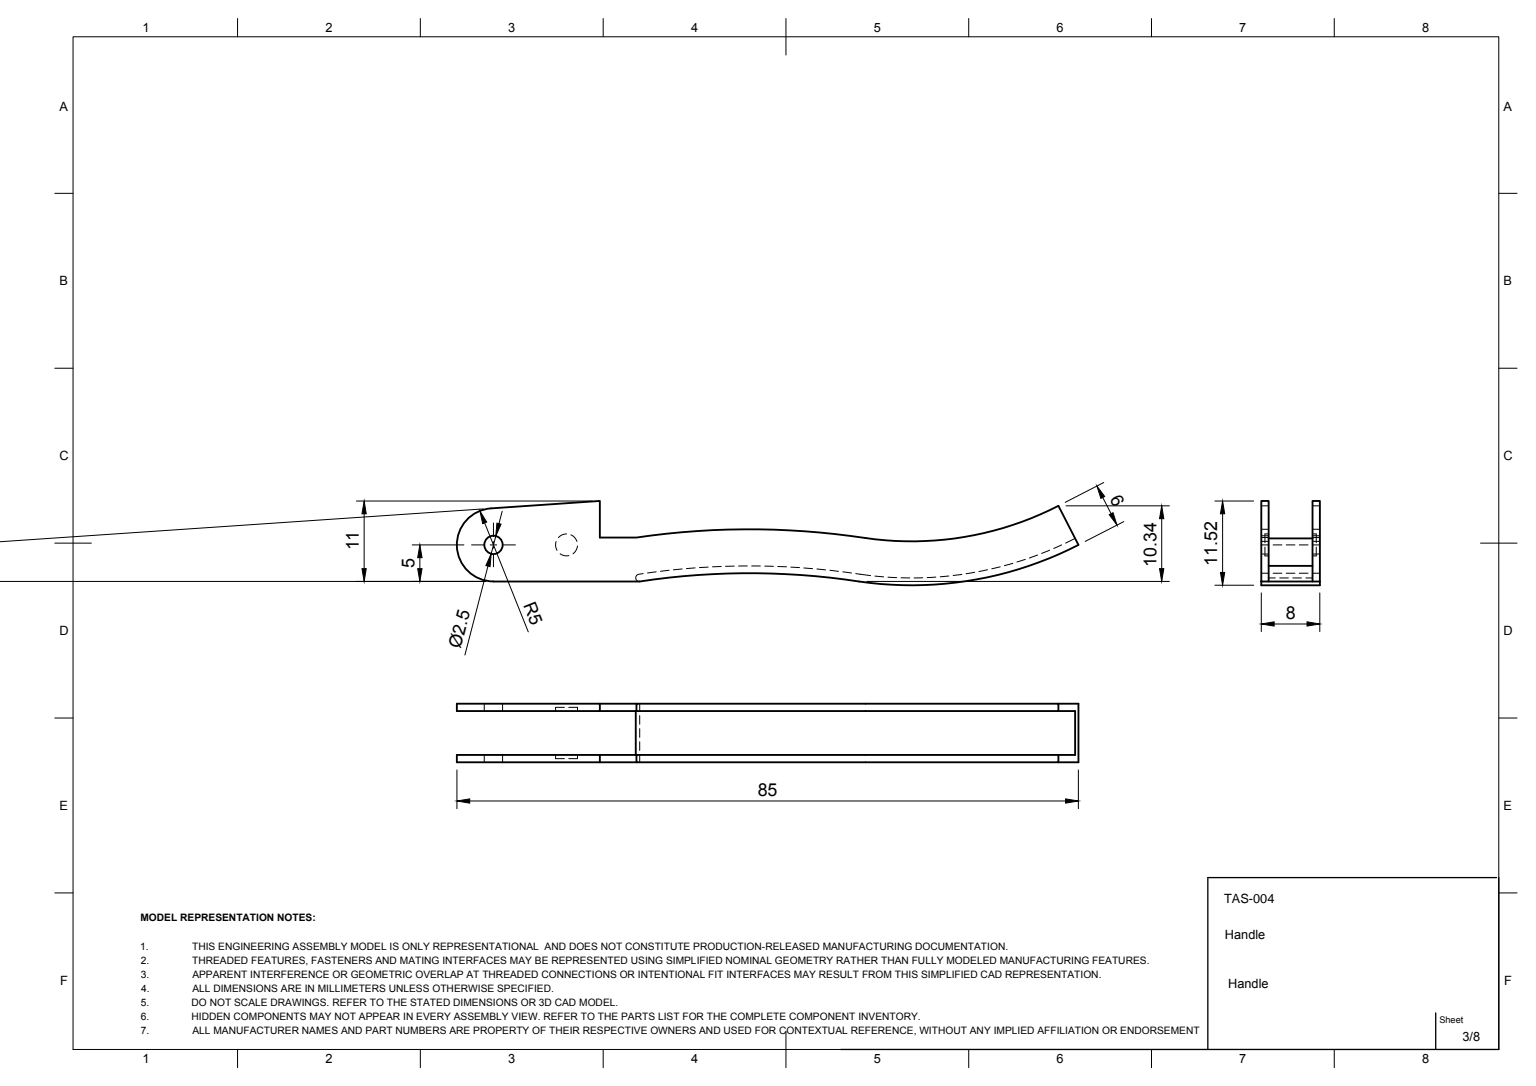
ISO-10303-21;
HEADER;
/* Generated by software containing ST-Developer
 * from STEP Tools, Inc. (www.steptools.com) 
 */

FILE_DESCRIPTION(
/* description */ ('STEP AP214'),
/* implementation_level */ '2;1');

FILE_NAME(
/* name */ 'Handle.step',
/* time_stamp */ '2026-11-04T19:48:07-08:00',
/* author */ (''),
/* organization */ (''),
/* preprocessor_version */ 'ST-DEVELOPER v20.2',
/* originating_system */ 'Autodesk Translation Framework v15.17.0.0',
/* authorisation */ '');

FILE_SCHEMA (('AUTOMOTIVE_DESIGN { 1 0 10303 214 3 1 1 }'));
ENDSEC;

DATA;
#10=MECHANICAL_DESIGN_GEOMETRIC_PRESENTATION_REPRESENTATION('',(#59),#9561);
#47=SHAPE_REPRESENTATION_RELATIONSHIP('SRR','None',#9587,#53);
#53=ADVANCED_BREP_SHAPE_REPRESENTATION('',(#65),#9555);
#59=STYLED_ITEM('',(#9626),#65);
#65=MANIFOLD_SOLID_BREP('Body1',#2405);
#71=FACE_BOUND('',#359,.T.);
#72=FACE_BOUND('',#361,.T.);
#73=FACE_BOUND('',#364,.T.);
#74=FACE_BOUND('',#365,.T.);
#75=FACE_BOUND('',#367,.T.);
#76=FACE_BOUND('',#368,.T.);
#86=PLANE('',#2504);
#87=PLANE('',#2505);
#88=PLANE('',#2509);
#89=PLANE('',#2510);
#90=PLANE('',#2514);
#91=PLANE('',#2515);
#92=PLANE('',#2516);
#93=PLANE('',#2526);
#94=PLANE('',#2527);
#95=PLANE('',#2528);
#96=PLANE('',#2532);
#97=PLANE('',#2534);
#98=PLANE('',#2537);
#99=PLANE('',#2538);
#194=FACE_OUTER_BOUND('',#337,.T.);
#195=FACE_OUTER_BOUND('',#338,.T.);
#196=FACE_OUTER_BOUND('',#339,.T.);
#197=FACE_OUTER_BOUND('',#340,.T.);
#198=FACE_OUTER_BOUND('',#341,.T.);
#199=FACE_OUTER_BOUND('',#342,.T.);
#200=FACE_OUTER_BOUND('',#343,.T.);
#201=FACE_OUTER_BOUND('',#344,.T.);
#202=FACE_OUTER_BOUND('',#345,.T.);
#203=FACE_OUTER_BOUND('',#346,.T.);
#204=FACE_OUTER_BOUND('',#347,.T.);
#205=FACE_OUTER_BOUND('',#348,.T.);
#206=FACE_OUTER_BOUND('',#349,.T.);
#207=FACE_OUTER_BOUND('',#350,.T.);
#208=FACE_OUTER_BOUND('',#351,.T.);
#209=FACE_OUTER_BOUND('',#352,.T.);
#210=FACE_OUTER_BOUND('',#353,.T.);
#211=FACE_OUTER_BOUND('',#354,.T.);
#212=FACE_OUTER_BOUND('',#355,.T.);
#213=FACE_OUTER_BOUND('',#356,.T.);
#214=FACE_OUTER_BOUND('',#357,.T.);
#215=FACE_OUTER_BOUND('',#358,.T.);
#216=FACE_OUTER_BOUND('',#360,.T.);
#217=FACE_OUTER_BOUND('',#362,.T.);
#218=FACE_OUTER_BOUND('',#363,.T.);
#219=FACE_OUTER_BOUND('',#366,.T.);
#220=FACE_OUTER_BOUND('',#369,.T.);
#221=FACE_OUTER_BOUND('',#370,.T.);
#222=FACE_OUTER_BOUND('',#371,.T.);
#337=EDGE_LOOP('',(#1583,#1584,#1585,#1586));
#338=EDGE_LOOP('',(#1587,#1588,#1589,#1590));
#339=EDGE_LOOP('',(#1591,#1592,#1593,#1594));
#340=EDGE_LOOP('',(#1595,#1596,#1597,#1598));
#341=EDGE_LOOP('',(#1599,#1600,#1601,#1602));
#342=EDGE_LOOP('',(#1603,#1604,#1605,#1606));
#343=EDGE_LOOP('',(#1607,#1608,#1609,#1610));
#344=EDGE_LOOP('',(#1611,#1612,#1613,#1614));
#345=EDGE_LOOP('',(#1615,#1616,#1617,#1618));
#346=EDGE_LOOP('',(#1619,#1620,#1621,#1622));
#347=EDGE_LOOP('',(#1623,#1624,#1625,#1626));
#348=EDGE_LOOP('',(#1627,#1628,#1629,#1630,#1631,#1632,#1633,#1634));
#349=EDGE_LOOP('',(#1635,#1636,#1637,#1638,#1639,#1640,#1641,#1642));
#350=EDGE_LOOP('',(#1643,#1644,#1645,#1646));
#351=EDGE_LOOP('',(#1647,#1648,#1649,#1650));
#352=EDGE_LOOP('',(#1651,#1652,#1653,#1654));
#353=EDGE_LOOP('',(#1655,#1656,#1657,#1658));
#354=EDGE_LOOP('',(#1659,#1660,#1661,#1662));
#355=EDGE_LOOP('',(#1663,#1664,#1665,#1666));
#356=EDGE_LOOP('',(#1667,#1668,#1669,#1670));
#357=EDGE_LOOP('',(#1671,#1672,#1673,#1674));
#358=EDGE_LOOP('',(#1675,#1676,#1677,#1678,#1679,#1680,#1681,#1682,#1683,
#1684));
#359=EDGE_LOOP('',(#1685));
#360=EDGE_LOOP('',(#1686,#1687,#1688,#1689,#1690,#1691,#1692,#1693,#1694,
#1695));
#361=EDGE_LOOP('',(#1696));
#362=EDGE_LOOP('',(#1697,#1698,#1699,#1700));
#363=EDGE_LOOP('',(#1701,#1702,#1703,#1704,#1705,#1706,#1707,#1708,#1709,
#1710,#1711));
#364=EDGE_LOOP('',(#1712));
#365=EDGE_LOOP('',(#1713));
#366=EDGE_LOOP('',(#1714,#1715,#1716,#1717,#1718,#1719,#1720,#1721,#1722,
#1723,#1724));
#367=EDGE_LOOP('',(#1725));
#368=EDGE_LOOP('',(#1726));
#369=EDGE_LOOP('',(#1727,#1728,#1729,#1730));
#370=EDGE_LOOP('',(#1731));
#371=EDGE_LOOP('',(#1732));
#495=LINE('',#3388,#745);
#496=LINE('',#3394,#746);
#497=LINE('',#3400,#747);
#498=LINE('',#3406,#748);
#499=LINE('',#3413,#749);
#500=LINE('',#3416,#750);
#501=LINE('',#3422,#751);
#502=LINE('',#3425,#752);
#503=LINE('',#3431,#753);
#504=LINE('',#3434,#754);
#505=LINE('',#3440,#755);
#506=LINE('',#3443,#756);
#507=LINE('',#3447,#757);
#508=LINE('',#3449,#758);
#509=LINE('',#3451,#759);
#510=LINE('',#3452,#760);
#511=LINE('',#3455,#761);
#512=LINE('',#3457,#762);
#513=LINE('',#3458,#763);
#514=LINE('',#3464,#764);
#515=LINE('',#3468,#765);
#516=LINE('',#3469,#766);
#517=LINE('',#3471,#767);
#518=LINE('',#3473,#768);
#519=LINE('',#3475,#769);
#520=LINE('',#3477,#770);
#521=LINE('',#3478,#771);
#522=LINE('',#3480,#772);
#523=LINE('',#3481,#773);
#524=LINE('',#3482,#774);
#525=LINE('',#3483,#775);
#526=LINE('',#3489,#776);
#527=LINE('',#3491,#777);
#528=LINE('',#3492,#778);
#529=LINE('',#3496,#779);
#530=LINE('',#3498,#780);
#531=LINE('',#3500,#781);
#532=LINE('',#3501,#782);
#533=LINE('',#3504,#783);
#534=LINE('',#3506,#784);
#535=LINE('',#3507,#785);
#536=LINE('',#3518,#786);
#537=LINE('',#3521,#787);
#538=LINE('',#3522,#788);
#539=LINE('',#3529,#789);
#745=VECTOR('',#2704,1.25);
#746=VECTOR('',#2711,1.25);
#747=VECTOR('',#2718,1.5);
#748=VECTOR('',#2725,1.5);
#749=VECTOR('',#2732,1000.);
#750=VECTOR('',#2735,1000.);
#751=VECTOR('',#2740,1000.);
#752=VECTOR('',#2743,1000.);
#753=VECTOR('',#2748,1000.);
#754=VECTOR('',#2751,1000.);
#755=VECTOR('',#2756,1000.);
#756=VECTOR('',#2759,1000.);
#757=VECTOR('',#2762,1000.);
#758=VECTOR('',#2763,1000.);
#759=VECTOR('',#2764,1000.);
#760=VECTOR('',#2765,1000.);
#761=VECTOR('',#2768,1000.);
#762=VECTOR('',#2769,1000.);
#763=VECTOR('',#2770,1000.);
#764=VECTOR('',#2777,1000.);
#765=VECTOR('',#2780,1000.);
#766=VECTOR('',#2781,1000.);
#767=VECTOR('',#2782,1000.);
#768=VECTOR('',#2783,1000.);
#769=VECTOR('',#2784,1000.);
#770=VECTOR('',#2785,1000.);
#771=VECTOR('',#2786,1000.);
#772=VECTOR('',#2789,1000.);
#773=VECTOR('',#2790,1000.);
#774=VECTOR('',#2791,1000.);
#775=VECTOR('',#2792,1000.);
#776=VECTOR('',#2799,1000.);
#777=VECTOR('',#2802,1000.);
#778=VECTOR('',#2803,1000.);
#779=VECTOR('',#2806,1000.);
#780=VECTOR('',#2807,1000.);
#781=VECTOR('',#2808,1000.);
#782=VECTOR('',#2809,1000.);
#783=VECTOR('',#2812,1000.);
#784=VECTOR('',#2813,1000.);
#785=VECTOR('',#2814,1000.);
#786=VECTOR('',#2831,1000.);
#787=VECTOR('',#2836,1000.);
#788=VECTOR('',#2837,1000.);
#789=VECTOR('',#2846,1000.);
#995=CIRCLE('',#2481,1.25);
#996=CIRCLE('',#2482,1.25);
#997=CIRCLE('',#2484,1.25);
#998=CIRCLE('',#2485,1.25);
#999=CIRCLE('',#2487,1.5);
#1000=CIRCLE('',#2488,1.5);
#1001=CIRCLE('',#2490,1.5);
#1002=CIRCLE('',#2491,1.5);
#1003=CIRCLE('',#2493,49.);
#1004=CIRCLE('',#2494,49.);
#1005=CIRCLE('',#2496,44.);
#1006=CIRCLE('',#2497,44.);
#1007=CIRCLE('',#2499,50.);
#1008=CIRCLE('',#2500,50.);
#1009=CIRCLE('',#2502,44.);
#1010=CIRCLE('',#2503,44.);
#1011=CIRCLE('',#2507,4.99999999999999);
#1012=CIRCLE('',#2508,4.99999999999999);
#1013=CIRCLE('',#2512,106.);
#1014=CIRCLE('',#2513,106.);
#1015=CIRCLE('',#2518,4.99999999999999);
#1016=CIRCLE('',#2519,4.99999999999999);
#1017=CIRCLE('',#2521,100.);
#1018=CIRCLE('',#2522,100.);
#1019=CIRCLE('',#2524,106.);
#1020=CIRCLE('',#2525,106.);
#1021=CIRCLE('',#2530,101.);
#1022=CIRCLE('',#2531,101.);
#1023=CIRCLE('',#2533,0.5);
#1024=CIRCLE('',#2535,0.5);
#1061=VERTEX_POINT('',#3385);
#1062=VERTEX_POINT('',#3387);
#1063=VERTEX_POINT('',#3391);
#1064=VERTEX_POINT('',#3393);
#1065=VERTEX_POINT('',#3397);
#1066=VERTEX_POINT('',#3399);
#1067=VERTEX_POINT('',#3403);
#1068=VERTEX_POINT('',#3405);
#1069=VERTEX_POINT('',#3409);
#1070=VERTEX_POINT('',#3410);
#1071=VERTEX_POINT('',#3412);
#1072=VERTEX_POINT('',#3414);
#1073=VERTEX_POINT('',#3418);
#1074=VERTEX_POINT('',#3419);
#1075=VERTEX_POINT('',#3421);
#1076=VERTEX_POINT('',#3423);
#1077=VERTEX_POINT('',#3427);
#1078=VERTEX_POINT('',#3428);
#1079=VERTEX_POINT('',#3430);
#1080=VERTEX_POINT('',#3432);
#1081=VERTEX_POINT('',#3436);
#1082=VERTEX_POINT('',#3437);
#1083=VERTEX_POINT('',#3439);
#1084=VERTEX_POINT('',#3441);
#1085=VERTEX_POINT('',#3445);
#1086=VERTEX_POINT('',#3446);
#1087=VERTEX_POINT('',#3448);
#1088=VERTEX_POINT('',#3450);
#1089=VERTEX_POINT('',#3454);
#1090=VERTEX_POINT('',#3456);
#1091=VERTEX_POINT('',#3460);
#1092=VERTEX_POINT('',#3462);
#1093=VERTEX_POINT('',#3466);
#1094=VERTEX_POINT('',#3467);
#1095=VERTEX_POINT('',#3470);
#1096=VERTEX_POINT('',#3472);
#1097=VERTEX_POINT('',#3474);
#1098=VERTEX_POINT('',#3476);
#1099=VERTEX_POINT('',#3485);
#1100=VERTEX_POINT('',#3487);
#1101=VERTEX_POINT('',#3494);
#1102=VERTEX_POINT('',#3495);
#1103=VERTEX_POINT('',#3497);
#1104=VERTEX_POINT('',#3499);
#1105=VERTEX_POINT('',#3503);
#1106=VERTEX_POINT('',#3505);
#1107=VERTEX_POINT('',#3515);
#1108=VERTEX_POINT('',#3517);
#1109=VERTEX_POINT('',#3526);
#1110=VERTEX_POINT('',#3528);
#1259=EDGE_CURVE('',#1061,#1061,#995,.T.);
#1260=EDGE_CURVE('',#1061,#1062,#495,.T.);
#1261=EDGE_CURVE('',#1062,#1062,#996,.T.);
#1262=EDGE_CURVE('',#1063,#1063,#997,.T.);
#1263=EDGE_CURVE('',#1063,#1064,#496,.T.);
#1264=EDGE_CURVE('',#1064,#1064,#998,.T.);
#1265=EDGE_CURVE('',#1065,#1065,#999,.T.);
#1266=EDGE_CURVE('',#1065,#1066,#497,.T.);
#1267=EDGE_CURVE('',#1066,#1066,#1000,.T.);
#1268=EDGE_CURVE('',#1067,#1067,#1001,.T.);
#1269=EDGE_CURVE('',#1067,#1068,#498,.T.);
#1270=EDGE_CURVE('',#1068,#1068,#1002,.T.);
#1271=EDGE_CURVE('',#1069,#1070,#1003,.T.);
#1272=EDGE_CURVE('',#1069,#1071,#499,.T.);
#1273=EDGE_CURVE('',#1071,#1072,#1004,.T.);
#1274=EDGE_CURVE('',#1070,#1072,#500,.T.);
#1275=EDGE_CURVE('',#1073,#1074,#1005,.T.);
#1276=EDGE_CURVE('',#1073,#1075,#501,.T.);
#1277=EDGE_CURVE('',#1075,#1076,#1006,.T.);
#1278=EDGE_CURVE('',#1074,#1076,#502,.T.);
#1279=EDGE_CURVE('',#1077,#1078,#1007,.T.);
#1280=EDGE_CURVE('',#1078,#1079,#503,.T.);
#1281=EDGE_CURVE('',#1080,#1079,#1008,.T.);
#1282=EDGE_CURVE('',#1077,#1080,#504,.T.);
#1283=EDGE_CURVE('',#1081,#1082,#1009,.T.);
#1284=EDGE_CURVE('',#1081,#1083,#505,.T.);
#1285=EDGE_CURVE('',#1083,#1084,#1010,.T.);
#1286=EDGE_CURVE('',#1082,#1084,#506,.T.);
#1287=EDGE_CURVE('',#1085,#1086,#507,.T.);
#1288=EDGE_CURVE('',#1085,#1087,#508,.T.);
#1289=EDGE_CURVE('',#1087,#1088,#509,.T.);
#1290=EDGE_CURVE('',#1086,#1088,#510,.T.);
#1291=EDGE_CURVE('',#1086,#1089,#511,.T.);
#1292=EDGE_CURVE('',#1088,#1090,#512,.T.);
#1293=EDGE_CURVE('',#1089,#1090,#513,.T.);
#1294=EDGE_CURVE('',#1089,#1091,#1011,.T.);
#1295=EDGE_CURVE('',#1090,#1092,#1012,.T.);
#1296=EDGE_CURVE('',#1091,#1092,#514,.T.);
#1297=EDGE_CURVE('',#1093,#1094,#515,.T.);
#1298=EDGE_CURVE('',#1094,#1091,#516,.T.);
#1299=EDGE_CURVE('',#1095,#1092,#517,.T.);
#1300=EDGE_CURVE('',#1096,#1095,#518,.T.);
#1301=EDGE_CURVE('',#1096,#1097,#519,.T.);
#1302=EDGE_CURVE('',#1097,#1098,#520,.T.);
#1303=EDGE_CURVE('',#1093,#1098,#521,.T.);
#1304=EDGE_CURVE('',#1071,#1081,#522,.T.);
#1305=EDGE_CURVE('',#1069,#1075,#523,.T.);
#1306=EDGE_CURVE('',#1077,#1073,#524,.T.);
#1307=EDGE_CURVE('',#1080,#1083,#525,.T.);
#1308=EDGE_CURVE('',#1082,#1099,#1013,.T.);
#1309=EDGE_CURVE('',#1084,#1100,#1014,.T.);
#1310=EDGE_CURVE('',#1099,#1100,#526,.T.);
#1311=EDGE_CURVE('',#1099,#1085,#527,.T.);
#1312=EDGE_CURVE('',#1100,#1087,#528,.T.);
#1313=EDGE_CURVE('',#1101,#1102,#529,.T.);
#1314=EDGE_CURVE('',#1102,#1103,#530,.T.);
#1315=EDGE_CURVE('',#1104,#1103,#531,.T.);
#1316=EDGE_CURVE('',#1101,#1104,#532,.T.);
#1317=EDGE_CURVE('',#1103,#1105,#533,.T.);
#1318=EDGE_CURVE('',#1106,#1105,#534,.T.);
#1319=EDGE_CURVE('',#1104,#1106,#535,.T.);
#1320=EDGE_CURVE('',#1105,#1098,#1015,.T.);
#1321=EDGE_CURVE('',#1106,#1097,#1016,.T.);
#1322=EDGE_CURVE('',#1079,#1095,#1017,.T.);
#1323=EDGE_CURVE('',#1078,#1096,#1018,.T.);
#1324=EDGE_CURVE('',#1076,#1107,#1019,.T.);
#1325=EDGE_CURVE('',#1108,#1107,#536,.T.);
#1326=EDGE_CURVE('',#1074,#1108,#1020,.T.);
#1327=EDGE_CURVE('',#1107,#1102,#537,.T.);
#1328=EDGE_CURVE('',#1108,#1101,#538,.T.);
#1329=EDGE_CURVE('',#1072,#1109,#1021,.T.);
#1330=EDGE_CURVE('',#1109,#1110,#539,.T.);
#1331=EDGE_CURVE('',#1070,#1110,#1022,.T.);
#1332=EDGE_CURVE('',#1110,#1093,#1023,.T.);
#1333=EDGE_CURVE('',#1094,#1109,#1024,.T.);
#1583=ORIENTED_EDGE('',*,*,#1259,.F.);
#1584=ORIENTED_EDGE('',*,*,#1260,.T.);
#1585=ORIENTED_EDGE('',*,*,#1261,.T.);
#1586=ORIENTED_EDGE('',*,*,#1260,.F.);
#1587=ORIENTED_EDGE('',*,*,#1262,.F.);
#1588=ORIENTED_EDGE('',*,*,#1263,.T.);
#1589=ORIENTED_EDGE('',*,*,#1264,.T.);
#1590=ORIENTED_EDGE('',*,*,#1263,.F.);
#1591=ORIENTED_EDGE('',*,*,#1265,.F.);
#1592=ORIENTED_EDGE('',*,*,#1266,.T.);
#1593=ORIENTED_EDGE('',*,*,#1267,.T.);
#1594=ORIENTED_EDGE('',*,*,#1266,.F.);
#1595=ORIENTED_EDGE('',*,*,#1268,.F.);
#1596=ORIENTED_EDGE('',*,*,#1269,.T.);
#1597=ORIENTED_EDGE('',*,*,#1270,.T.);
#1598=ORIENTED_EDGE('',*,*,#1269,.F.);
#1599=ORIENTED_EDGE('',*,*,#1271,.F.);
#1600=ORIENTED_EDGE('',*,*,#1272,.T.);
#1601=ORIENTED_EDGE('',*,*,#1273,.T.);
#1602=ORIENTED_EDGE('',*,*,#1274,.F.);
#1603=ORIENTED_EDGE('',*,*,#1275,.F.);
#1604=ORIENTED_EDGE('',*,*,#1276,.T.);
#1605=ORIENTED_EDGE('',*,*,#1277,.T.);
#1606=ORIENTED_EDGE('',*,*,#1278,.F.);
#1607=ORIENTED_EDGE('',*,*,#1279,.T.);
#1608=ORIENTED_EDGE('',*,*,#1280,.T.);
#1609=ORIENTED_EDGE('',*,*,#1281,.F.);
#1610=ORIENTED_EDGE('',*,*,#1282,.F.);
#1611=ORIENTED_EDGE('',*,*,#1283,.F.);
#1612=ORIENTED_EDGE('',*,*,#1284,.T.);
#1613=ORIENTED_EDGE('',*,*,#1285,.T.);
#1614=ORIENTED_EDGE('',*,*,#1286,.F.);
#1615=ORIENTED_EDGE('',*,*,#1287,.F.);
#1616=ORIENTED_EDGE('',*,*,#1288,.T.);
#1617=ORIENTED_EDGE('',*,*,#1289,.T.);
#1618=ORIENTED_EDGE('',*,*,#1290,.F.);
#1619=ORIENTED_EDGE('',*,*,#1291,.F.);
#1620=ORIENTED_EDGE('',*,*,#1290,.T.);
#1621=ORIENTED_EDGE('',*,*,#1292,.T.);
#1622=ORIENTED_EDGE('',*,*,#1293,.F.);
#1623=ORIENTED_EDGE('',*,*,#1294,.F.);
#1624=ORIENTED_EDGE('',*,*,#1293,.T.);
#1625=ORIENTED_EDGE('',*,*,#1295,.T.);
#1626=ORIENTED_EDGE('',*,*,#1296,.F.);
#1627=ORIENTED_EDGE('',*,*,#1297,.T.);
#1628=ORIENTED_EDGE('',*,*,#1298,.T.);
#1629=ORIENTED_EDGE('',*,*,#1296,.T.);
#1630=ORIENTED_EDGE('',*,*,#1299,.F.);
#1631=ORIENTED_EDGE('',*,*,#1300,.F.);
#1632=ORIENTED_EDGE('',*,*,#1301,.T.);
#1633=ORIENTED_EDGE('',*,*,#1302,.T.);
#1634=ORIENTED_EDGE('',*,*,#1303,.F.);
#1635=ORIENTED_EDGE('',*,*,#1304,.F.);
#1636=ORIENTED_EDGE('',*,*,#1272,.F.);
#1637=ORIENTED_EDGE('',*,*,#1305,.T.);
#1638=ORIENTED_EDGE('',*,*,#1276,.F.);
#1639=ORIENTED_EDGE('',*,*,#1306,.F.);
#1640=ORIENTED_EDGE('',*,*,#1282,.T.);
#1641=ORIENTED_EDGE('',*,*,#1307,.T.);
#1642=ORIENTED_EDGE('',*,*,#1284,.F.);
#1643=ORIENTED_EDGE('',*,*,#1308,.F.);
#1644=ORIENTED_EDGE('',*,*,#1286,.T.);
#1645=ORIENTED_EDGE('',*,*,#1309,.T.);
#1646=ORIENTED_EDGE('',*,*,#1310,.F.);
#1647=ORIENTED_EDGE('',*,*,#1311,.F.);
#1648=ORIENTED_EDGE('',*,*,#1310,.T.);
#1649=ORIENTED_EDGE('',*,*,#1312,.T.);
#1650=ORIENTED_EDGE('',*,*,#1288,.F.);
#1651=ORIENTED_EDGE('',*,*,#1313,.T.);
#1652=ORIENTED_EDGE('',*,*,#1314,.T.);
#1653=ORIENTED_EDGE('',*,*,#1315,.F.);
#1654=ORIENTED_EDGE('',*,*,#1316,.F.);
#1655=ORIENTED_EDGE('',*,*,#1315,.T.);
#1656=ORIENTED_EDGE('',*,*,#1317,.T.);
#1657=ORIENTED_EDGE('',*,*,#1318,.F.);
#1658=ORIENTED_EDGE('',*,*,#1319,.F.);
#1659=ORIENTED_EDGE('',*,*,#1318,.T.);
#1660=ORIENTED_EDGE('',*,*,#1320,.T.);
#1661=ORIENTED_EDGE('',*,*,#1302,.F.);
#1662=ORIENTED_EDGE('',*,*,#1321,.F.);
#1663=ORIENTED_EDGE('',*,*,#1322,.F.);
#1664=ORIENTED_EDGE('',*,*,#1280,.F.);
#1665=ORIENTED_EDGE('',*,*,#1323,.T.);
#1666=ORIENTED_EDGE('',*,*,#1300,.T.);
#1667=ORIENTED_EDGE('',*,*,#1278,.T.);
#1668=ORIENTED_EDGE('',*,*,#1324,.T.);
#1669=ORIENTED_EDGE('',*,*,#1325,.F.);
#1670=ORIENTED_EDGE('',*,*,#1326,.F.);
#1671=ORIENTED_EDGE('',*,*,#1325,.T.);
#1672=ORIENTED_EDGE('',*,*,#1327,.T.);
#1673=ORIENTED_EDGE('',*,*,#1313,.F.);
#1674=ORIENTED_EDGE('',*,*,#1328,.F.);
#1675=ORIENTED_EDGE('',*,*,#1316,.T.);
#1676=ORIENTED_EDGE('',*,*,#1319,.T.);
#1677=ORIENTED_EDGE('',*,*,#1321,.T.);
#1678=ORIENTED_EDGE('',*,*,#1301,.F.);
#1679=ORIENTED_EDGE('',*,*,#1323,.F.);
#1680=ORIENTED_EDGE('',*,*,#1279,.F.);
#1681=ORIENTED_EDGE('',*,*,#1306,.T.);
#1682=ORIENTED_EDGE('',*,*,#1275,.T.);
#1683=ORIENTED_EDGE('',*,*,#1326,.T.);
#1684=ORIENTED_EDGE('',*,*,#1328,.T.);
#1685=ORIENTED_EDGE('',*,*,#1261,.F.);
#1686=ORIENTED_EDGE('',*,*,#1289,.F.);
#1687=ORIENTED_EDGE('',*,*,#1312,.F.);
#1688=ORIENTED_EDGE('',*,*,#1309,.F.);
#1689=ORIENTED_EDGE('',*,*,#1285,.F.);
#1690=ORIENTED_EDGE('',*,*,#1307,.F.);
#1691=ORIENTED_EDGE('',*,*,#1281,.T.);
#1692=ORIENTED_EDGE('',*,*,#1322,.T.);
#1693=ORIENTED_EDGE('',*,*,#1299,.T.);
#1694=ORIENTED_EDGE('',*,*,#1295,.F.);
#1695=ORIENTED_EDGE('',*,*,#1292,.F.);
#1696=ORIENTED_EDGE('',*,*,#1262,.T.);
#1697=ORIENTED_EDGE('',*,*,#1329,.T.);
#1698=ORIENTED_EDGE('',*,*,#1330,.T.);
#1699=ORIENTED_EDGE('',*,*,#1331,.F.);
#1700=ORIENTED_EDGE('',*,*,#1274,.T.);
#1701=ORIENTED_EDGE('',*,*,#1314,.F.);
#1702=ORIENTED_EDGE('',*,*,#1327,.F.);
#1703=ORIENTED_EDGE('',*,*,#1324,.F.);
#1704=ORIENTED_EDGE('',*,*,#1277,.F.);
#1705=ORIENTED_EDGE('',*,*,#1305,.F.);
#1706=ORIENTED_EDGE('',*,*,#1271,.T.);
#1707=ORIENTED_EDGE('',*,*,#1331,.T.);
#1708=ORIENTED_EDGE('',*,*,#1332,.T.);
#1709=ORIENTED_EDGE('',*,*,#1303,.T.);
#1710=ORIENTED_EDGE('',*,*,#1320,.F.);
#1711=ORIENTED_EDGE('',*,*,#1317,.F.);
#1712=ORIENTED_EDGE('',*,*,#1259,.T.);
#1713=ORIENTED_EDGE('',*,*,#1265,.T.);
#1714=ORIENTED_EDGE('',*,*,#1287,.T.);
#1715=ORIENTED_EDGE('',*,*,#1291,.T.);
#1716=ORIENTED_EDGE('',*,*,#1294,.T.);
#1717=ORIENTED_EDGE('',*,*,#1298,.F.);
#1718=ORIENTED_EDGE('',*,*,#1333,.T.);
#1719=ORIENTED_EDGE('',*,*,#1329,.F.);
#1720=ORIENTED_EDGE('',*,*,#1273,.F.);
#1721=ORIENTED_EDGE('',*,*,#1304,.T.);
#1722=ORIENTED_EDGE('',*,*,#1283,.T.);
#1723=ORIENTED_EDGE('',*,*,#1308,.T.);
#1724=ORIENTED_EDGE('',*,*,#1311,.T.);
#1725=ORIENTED_EDGE('',*,*,#1264,.F.);
#1726=ORIENTED_EDGE('',*,*,#1270,.F.);
#1727=ORIENTED_EDGE('',*,*,#1332,.F.);
#1728=ORIENTED_EDGE('',*,*,#1330,.F.);
#1729=ORIENTED_EDGE('',*,*,#1333,.F.);
#1730=ORIENTED_EDGE('',*,*,#1297,.F.);
#1731=ORIENTED_EDGE('',*,*,#1268,.T.);
#1732=ORIENTED_EDGE('',*,*,#1267,.F.);
#2231=CYLINDRICAL_SURFACE('',#2480,1.25);
#2232=CYLINDRICAL_SURFACE('',#2483,1.25);
#2233=CYLINDRICAL_SURFACE('',#2486,1.5);
#2234=CYLINDRICAL_SURFACE('',#2489,1.5);
#2235=CYLINDRICAL_SURFACE('',#2492,49.);
#2236=CYLINDRICAL_SURFACE('',#2495,44.);
#2237=CYLINDRICAL_SURFACE('',#2498,50.);
#2238=CYLINDRICAL_SURFACE('',#2501,44.);
#2239=CYLINDRICAL_SURFACE('',#2506,4.99999999999999);
#2240=CYLINDRICAL_SURFACE('',#2511,106.);
#2241=CYLINDRICAL_SURFACE('',#2517,4.99999999999999);
#2242=CYLINDRICAL_SURFACE('',#2520,100.);
#2243=CYLINDRICAL_SURFACE('',#2523,106.);
#2244=CYLINDRICAL_SURFACE('',#2529,101.);
#2245=CYLINDRICAL_SURFACE('',#2536,0.5);
#2262=ADVANCED_FACE('',(#194),#2231,.F.);
#2263=ADVANCED_FACE('',(#195),#2232,.F.);
#2264=ADVANCED_FACE('',(#196),#2233,.F.);
#2265=ADVANCED_FACE('',(#197),#2234,.F.);
#2266=ADVANCED_FACE('',(#198),#2235,.F.);
#2267=ADVANCED_FACE('',(#199),#2236,.F.);
#2268=ADVANCED_FACE('',(#200),#2237,.T.);
#2269=ADVANCED_FACE('',(#201),#2238,.F.);
#2270=ADVANCED_FACE('',(#202),#86,.F.);
#2271=ADVANCED_FACE('',(#203),#87,.F.);
#2272=ADVANCED_FACE('',(#204),#2239,.T.);
#2273=ADVANCED_FACE('',(#205),#88,.T.);
#2274=ADVANCED_FACE('',(#206),#89,.F.);
#2275=ADVANCED_FACE('',(#207),#2240,.T.);
#2276=ADVANCED_FACE('',(#208),#90,.F.);
#2277=ADVANCED_FACE('',(#209),#91,.F.);
#2278=ADVANCED_FACE('',(#210),#92,.F.);
#2279=ADVANCED_FACE('',(#211),#2241,.T.);
#2280=ADVANCED_FACE('',(#212),#2242,.F.);
#2281=ADVANCED_FACE('',(#213),#2243,.T.);
#2282=ADVANCED_FACE('',(#214),#93,.F.);
#2283=ADVANCED_FACE('',(#215,#71),#94,.T.);
#2284=ADVANCED_FACE('',(#216,#72),#95,.F.);
#2285=ADVANCED_FACE('',(#217),#2244,.T.);
#2286=ADVANCED_FACE('',(#218,#73,#74),#96,.F.);
#2287=ADVANCED_FACE('',(#219,#75,#76),#97,.T.);
#2288=ADVANCED_FACE('',(#220),#2245,.T.);
#2289=ADVANCED_FACE('',(#221),#98,.T.);
#2290=ADVANCED_FACE('',(#222),#99,.F.);
#2405=CLOSED_SHELL('',(#2262,#2263,#2264,#2265,#2266,#2267,#2268,#2269,
#2270,#2271,#2272,#2273,#2274,#2275,#2276,#2277,#2278,#2279,#2280,#2281,
#2282,#2283,#2284,#2285,#2286,#2287,#2288,#2289,#2290));
#2479=AXIS2_PLACEMENT_3D('',#3383,#2698,#2699);
#2480=AXIS2_PLACEMENT_3D('',#3384,#2700,#2701);
#2481=AXIS2_PLACEMENT_3D('',#3386,#2702,#2703);
#2482=AXIS2_PLACEMENT_3D('',#3389,#2705,#2706);
#2483=AXIS2_PLACEMENT_3D('',#3390,#2707,#2708);
#2484=AXIS2_PLACEMENT_3D('',#3392,#2709,#2710);
#2485=AXIS2_PLACEMENT_3D('',#3395,#2712,#2713);
#2486=AXIS2_PLACEMENT_3D('',#3396,#2714,#2715);
#2487=AXIS2_PLACEMENT_3D('',#3398,#2716,#2717);
#2488=AXIS2_PLACEMENT_3D('',#3401,#2719,#2720);
#2489=AXIS2_PLACEMENT_3D('',#3402,#2721,#2722);
#2490=AXIS2_PLACEMENT_3D('',#3404,#2723,#2724);
#2491=AXIS2_PLACEMENT_3D('',#3407,#2726,#2727);
#2492=AXIS2_PLACEMENT_3D('',#3408,#2728,#2729);
#2493=AXIS2_PLACEMENT_3D('',#3411,#2730,#2731);
#2494=AXIS2_PLACEMENT_3D('',#3415,#2733,#2734);
#2495=AXIS2_PLACEMENT_3D('',#3417,#2736,#2737);
#2496=AXIS2_PLACEMENT_3D('',#3420,#2738,#2739);
#2497=AXIS2_PLACEMENT_3D('',#3424,#2741,#2742);
#2498=AXIS2_PLACEMENT_3D('',#3426,#2744,#2745);
#2499=AXIS2_PLACEMENT_3D('',#3429,#2746,#2747);
#2500=AXIS2_PLACEMENT_3D('',#3433,#2749,#2750);
#2501=AXIS2_PLACEMENT_3D('',#3435,#2752,#2753);
#2502=AXIS2_PLACEMENT_3D('',#3438,#2754,#2755);
#2503=AXIS2_PLACEMENT_3D('',#3442,#2757,#2758);
#2504=AXIS2_PLACEMENT_3D('',#3444,#2760,#2761);
#2505=AXIS2_PLACEMENT_3D('',#3453,#2766,#2767);
#2506=AXIS2_PLACEMENT_3D('',#3459,#2771,#2772);
#2507=AXIS2_PLACEMENT_3D('',#3461,#2773,#2774);
#2508=AXIS2_PLACEMENT_3D('',#3463,#2775,#2776);
#2509=AXIS2_PLACEMENT_3D('',#3465,#2778,#2779);
#2510=AXIS2_PLACEMENT_3D('',#3479,#2787,#2788);
#2511=AXIS2_PLACEMENT_3D('',#3484,#2793,#2794);
#2512=AXIS2_PLACEMENT_3D('',#3486,#2795,#2796);
#2513=AXIS2_PLACEMENT_3D('',#3488,#2797,#2798);
#2514=AXIS2_PLACEMENT_3D('',#3490,#2800,#2801);
#2515=AXIS2_PLACEMENT_3D('',#3493,#2804,#2805);
#2516=AXIS2_PLACEMENT_3D('',#3502,#2810,#2811);
#2517=AXIS2_PLACEMENT_3D('',#3508,#2815,#2816);
#2518=AXIS2_PLACEMENT_3D('',#3509,#2817,#2818);
#2519=AXIS2_PLACEMENT_3D('',#3510,#2819,#2820);
#2520=AXIS2_PLACEMENT_3D('',#3511,#2821,#2822);
#2521=AXIS2_PLACEMENT_3D('',#3512,#2823,#2824);
#2522=AXIS2_PLACEMENT_3D('',#3513,#2825,#2826);
#2523=AXIS2_PLACEMENT_3D('',#3514,#2827,#2828);
#2524=AXIS2_PLACEMENT_3D('',#3516,#2829,#2830);
#2525=AXIS2_PLACEMENT_3D('',#3519,#2832,#2833);
#2526=AXIS2_PLACEMENT_3D('',#3520,#2834,#2835);
#2527=AXIS2_PLACEMENT_3D('',#3523,#2838,#2839);
#2528=AXIS2_PLACEMENT_3D('',#3524,#2840,#2841);
#2529=AXIS2_PLACEMENT_3D('',#3525,#2842,#2843);
#2530=AXIS2_PLACEMENT_3D('',#3527,#2844,#2845);
#2531=AXIS2_PLACEMENT_3D('',#3530,#2847,#2848);
#2532=AXIS2_PLACEMENT_3D('',#3531,#2849,#2850);
#2533=AXIS2_PLACEMENT_3D('',#3532,#2851,#2852);
#2534=AXIS2_PLACEMENT_3D('',#3533,#2853,#2854);
#2535=AXIS2_PLACEMENT_3D('',#3534,#2855,#2856);
#2536=AXIS2_PLACEMENT_3D('',#3535,#2857,#2858);
#2537=AXIS2_PLACEMENT_3D('',#3536,#2859,#2860);
#2538=AXIS2_PLACEMENT_3D('',#3537,#2861,#2862);
#2698=DIRECTION('axis',(0.,0.,1.));
#2699=DIRECTION('refdir',(1.,0.,0.));
#2700=DIRECTION('center_axis',(0.,0.,1.));
#2701=DIRECTION('ref_axis',(1.,0.,0.));
#2702=DIRECTION('center_axis',(0.,0.,1.));
#2703=DIRECTION('ref_axis',(1.,0.,0.));
#2704=DIRECTION('',(0.,0.,1.));
#2705=DIRECTION('center_axis',(0.,0.,1.));
#2706=DIRECTION('ref_axis',(1.,0.,0.));
#2707=DIRECTION('center_axis',(0.,0.,1.));
#2708=DIRECTION('ref_axis',(1.,0.,0.));
#2709=DIRECTION('center_axis',(0.,0.,1.));
#2710=DIRECTION('ref_axis',(1.,0.,0.));
#2711=DIRECTION('',(0.,0.,1.));
#2712=DIRECTION('center_axis',(0.,0.,1.));
#2713=DIRECTION('ref_axis',(1.,0.,0.));
#2714=DIRECTION('center_axis',(0.,0.,1.));
#2715=DIRECTION('ref_axis',(1.,0.,0.));
#2716=DIRECTION('center_axis',(0.,0.,1.));
#2717=DIRECTION('ref_axis',(1.,0.,0.));
#2718=DIRECTION('',(0.,0.,1.));
#2719=DIRECTION('center_axis',(0.,0.,1.));
#2720=DIRECTION('ref_axis',(1.,0.,0.));
#2721=DIRECTION('center_axis',(0.,0.,1.));
#2722=DIRECTION('ref_axis',(1.,0.,0.));
#2723=DIRECTION('center_axis',(0.,0.,1.));
#2724=DIRECTION('ref_axis',(1.,0.,0.));
#2725=DIRECTION('',(0.,0.,1.));
#2726=DIRECTION('center_axis',(0.,0.,1.));
#2727=DIRECTION('ref_axis',(1.,0.,0.));
#2728=DIRECTION('center_axis',(0.,0.,-1.));
#2729=DIRECTION('ref_axis',(-1.,0.,0.));
#2730=DIRECTION('center_axis',(0.,0.,-1.));
#2731=DIRECTION('ref_axis',(1.,0.,0.));
#2732=DIRECTION('',(0.,0.,-1.));
#2733=DIRECTION('center_axis',(0.,0.,-1.));
#2734=DIRECTION('ref_axis',(1.,0.,0.));
#2735=DIRECTION('',(0.,0.,-1.));
#2736=DIRECTION('center_axis',(0.,0.,-1.));
#2737=DIRECTION('ref_axis',(-1.,0.,0.));
#2738=DIRECTION('center_axis',(0.,0.,-1.));
#2739=DIRECTION('ref_axis',(-1.,0.,0.));
#2740=DIRECTION('',(0.,0.,-1.));
#2741=DIRECTION('center_axis',(0.,0.,-1.));
#2742=DIRECTION('ref_axis',(1.,0.,0.));
#2743=DIRECTION('',(0.,0.,-1.));
#2744=DIRECTION('center_axis',(0.,0.,-1.));
#2745=DIRECTION('ref_axis',(-1.,0.,0.));
#2746=DIRECTION('center_axis',(0.,0.,-1.));
#2747=DIRECTION('ref_axis',(-1.,0.,0.));
#2748=DIRECTION('',(0.,0.,-1.));
#2749=DIRECTION('center_axis',(0.,0.,-1.));
#2750=DIRECTION('ref_axis',(-1.,0.,0.));
#2751=DIRECTION('',(0.,0.,-1.));
#2752=DIRECTION('center_axis',(0.,0.,-1.));
#2753=DIRECTION('ref_axis',(-1.,0.,0.));
#2754=DIRECTION('center_axis',(0.,0.,-1.));
#2755=DIRECTION('ref_axis',(1.,0.,0.));
#2756=DIRECTION('',(0.,0.,-1.));
#2757=DIRECTION('center_axis',(0.,0.,-1.));
#2758=DIRECTION('ref_axis',(-1.,0.,0.));
#2759=DIRECTION('',(0.,0.,-1.));
#2760=DIRECTION('center_axis',(0.,1.,0.));
#2761=DIRECTION('ref_axis',(0.,0.,1.));
#2762=DIRECTION('',(1.,0.,0.));
#2763=DIRECTION('',(0.,0.,-1.));
#2764=DIRECTION('',(1.,0.,0.));
#2765=DIRECTION('',(0.,0.,-1.));
#2766=DIRECTION('center_axis',(-0.997701530936239,-0.0677617529841435,0.));
#2767=DIRECTION('ref_axis',(0.0677617529841435,-0.997701530936239,0.));
#2768=DIRECTION('',(-0.0677617529841435,0.997701530936239,0.));
#2769=DIRECTION('',(-0.0677617529841435,0.997701530936239,0.));
#2770=DIRECTION('',(0.,0.,-1.));
#2771=DIRECTION('center_axis',(0.,0.,-1.));
#2772=DIRECTION('ref_axis',(-1.,0.,0.));
#2773=DIRECTION('center_axis',(0.,0.,1.));
#2774=DIRECTION('ref_axis',(1.,0.,0.));
#2775=DIRECTION('center_axis',(0.,0.,1.));
#2776=DIRECTION('ref_axis',(1.,0.,0.));
#2777=DIRECTION('',(0.,0.,-1.));
#2778=DIRECTION('center_axis',(-1.,0.,0.));
#2779=DIRECTION('ref_axis',(0.,0.,1.));
#2780=DIRECTION('',(0.,0.,-1.));
#2781=DIRECTION('',(0.,1.,0.));
#2782=DIRECTION('',(0.,1.,0.));
#2783=DIRECTION('',(0.,0.,-1.));
#2784=DIRECTION('',(0.,1.,0.));
#2785=DIRECTION('',(0.,0.,-1.));
#2786=DIRECTION('',(0.,1.,0.));
#2787=DIRECTION('center_axis',(-0.456611069299162,0.889666415794974,0.));
#2788=DIRECTION('ref_axis',(-0.889666415794975,-0.456611069299162,0.));
#2789=DIRECTION('',(0.889666415794974,0.456611069299162,0.));
#2790=DIRECTION('',(0.889666415794974,0.456611069299162,0.));
#2791=DIRECTION('',(0.889666415794974,0.456611069299162,0.));
#2792=DIRECTION('',(0.889666415794974,0.456611069299162,0.));
#2793=DIRECTION('center_axis',(0.,0.,-1.));
#2794=DIRECTION('ref_axis',(0.999997864451694,-0.0020666620553607,0.));
#2795=DIRECTION('center_axis',(0.,0.,1.));
#2796=DIRECTION('ref_axis',(1.,0.,0.));
#2797=DIRECTION('center_axis',(0.,0.,1.));
#2798=DIRECTION('ref_axis',(1.,0.,0.));
#2799=DIRECTION('',(0.,0.,-1.));
#2800=DIRECTION('center_axis',(-1.,1.04083408558608E-15,0.));
#2801=DIRECTION('ref_axis',(-1.04083408558608E-15,-1.,0.));
#2802=DIRECTION('',(1.04083408558608E-15,1.,0.));
#2803=DIRECTION('',(1.04083408558608E-15,1.,0.));
#2804=DIRECTION('center_axis',(0.,1.,0.));
#2805=DIRECTION('ref_axis',(0.,0.,1.));
#2806=DIRECTION('',(0.,0.,-1.));
#2807=DIRECTION('',(1.,0.,0.));
#2808=DIRECTION('',(0.,0.,-1.));
#2809=DIRECTION('',(1.,0.,0.));
#2810=DIRECTION('center_axis',(-0.997701530936239,-0.0677617529841435,0.));
#2811=DIRECTION('ref_axis',(0.0677617529841435,-0.997701530936239,0.));
#2812=DIRECTION('',(-0.0677617529841435,0.997701530936239,0.));
#2813=DIRECTION('',(0.,0.,-1.));
#2814=DIRECTION('',(-0.0677617529841435,0.997701530936239,0.));
#2815=DIRECTION('center_axis',(0.,0.,-1.));
#2816=DIRECTION('ref_axis',(-1.,0.,0.));
#2817=DIRECTION('center_axis',(0.,0.,1.));
#2818=DIRECTION('ref_axis',(1.,0.,0.));
#2819=DIRECTION('center_axis',(0.,0.,1.));
#2820=DIRECTION('ref_axis',(1.,0.,0.));
#2821=DIRECTION('center_axis',(0.,0.,-1.));
#2822=DIRECTION('ref_axis',(1.,1.22464679914735E-16,0.));
#2823=DIRECTION('center_axis',(0.,0.,1.));
#2824=DIRECTION('ref_axis',(1.,0.,0.));
#2825=DIRECTION('center_axis',(0.,0.,1.));
#2826=DIRECTION('ref_axis',(1.,0.,0.));
#2827=DIRECTION('center_axis',(0.,0.,-1.));
#2828=DIRECTION('ref_axis',(0.999997864451694,-0.00206666205536139,0.));
#2829=DIRECTION('center_axis',(0.,0.,1.));
#2830=DIRECTION('ref_axis',(1.,0.,0.));
#2831=DIRECTION('',(0.,0.,-1.));
#2832=DIRECTION('center_axis',(0.,0.,1.));
#2833=DIRECTION('ref_axis',(1.,0.,0.));
#2834=DIRECTION('center_axis',(-1.,1.04083408558608E-15,0.));
#2835=DIRECTION('ref_axis',(-1.04083408558608E-15,-1.,0.));
#2836=DIRECTION('',(1.04083408558608E-15,1.,0.));
#2837=DIRECTION('',(1.04083408558608E-15,1.,0.));
#2838=DIRECTION('center_axis',(0.,0.,1.));
#2839=DIRECTION('ref_axis',(1.,0.,0.));
#2840=DIRECTION('center_axis',(0.,0.,1.));
#2841=DIRECTION('ref_axis',(1.,0.,0.));
#2842=DIRECTION('center_axis',(0.,0.,-1.));
#2843=DIRECTION('ref_axis',(0.999999985346409,-0.000171193403699097,0.));
#2844=DIRECTION('center_axis',(0.,0.,1.));
#2845=DIRECTION('ref_axis',(1.,0.,0.));
#2846=DIRECTION('',(0.,0.,1.));
#2847=DIRECTION('center_axis',(0.,0.,1.));
#2848=DIRECTION('ref_axis',(1.,0.,0.));
#2849=DIRECTION('center_axis',(0.,0.,1.));
#2850=DIRECTION('ref_axis',(1.,0.,0.));
#2851=DIRECTION('center_axis',(0.,0.,1.));
#2852=DIRECTION('ref_axis',(1.,0.,0.));
#2853=DIRECTION('center_axis',(0.,0.,1.));
#2854=DIRECTION('ref_axis',(1.,0.,0.));
#2855=DIRECTION('center_axis',(0.,0.,-1.));
#2856=DIRECTION('ref_axis',(1.,0.,0.));
#2857=DIRECTION('center_axis',(0.,0.,-1.));
#2858=DIRECTION('ref_axis',(-1.,0.,0.));
#2859=DIRECTION('center_axis',(0.,0.,1.));
#2860=DIRECTION('ref_axis',(1.,0.,0.));
#2861=DIRECTION('center_axis',(0.,0.,1.));
#2862=DIRECTION('ref_axis',(1.,0.,0.));
#3383=CARTESIAN_POINT('',(0.,0.,0.));
#3384=CARTESIAN_POINT('Origin',(0.,0.,-4.5));
#3385=CARTESIAN_POINT('',(-1.25,-1.53080849893419E-16,3.));
#3386=CARTESIAN_POINT('Origin',(0.,0.,3.));
#3387=CARTESIAN_POINT('',(-1.25,-1.53080849893419E-16,4.));
#3388=CARTESIAN_POINT('',(-1.25,-1.53080849893419E-16,-4.5));
#3389=CARTESIAN_POINT('Origin',(0.,0.,4.));
#3390=CARTESIAN_POINT('Origin',(0.,0.,-4.5));
#3391=CARTESIAN_POINT('',(-1.25,-1.53080849893419E-16,-4.));
#3392=CARTESIAN_POINT('Origin',(0.,0.,-4.));
#3393=CARTESIAN_POINT('',(-1.25,-1.53080849893419E-16,-3.));
#3394=CARTESIAN_POINT('',(-1.25,-1.53080849893419E-16,-4.5));
#3395=CARTESIAN_POINT('Origin',(0.,0.,-3.));
#3396=CARTESIAN_POINT('Origin',(0.,-10.,-3.5));
#3397=CARTESIAN_POINT('',(-1.5,-10.,3.));
#3398=CARTESIAN_POINT('Origin',(0.,-10.,3.));
#3399=CARTESIAN_POINT('',(-1.5,-10.,3.5));
#3400=CARTESIAN_POINT('',(-1.5,-10.,-3.5));
#3401=CARTESIAN_POINT('Origin',(0.,-10.,3.5));
#3402=CARTESIAN_POINT('Origin',(0.,-10.,-3.5));
#3403=CARTESIAN_POINT('',(-1.5,-10.,-3.5));
#3404=CARTESIAN_POINT('Origin',(0.,-10.,-3.5));
#3405=CARTESIAN_POINT('',(-1.5,-10.,-3.));
#3406=CARTESIAN_POINT('',(-1.5,-10.,-3.5));
#3407=CARTESIAN_POINT('Origin',(0.,-10.,-3.));
#3408=CARTESIAN_POINT('Origin',(44.4833207897487,-57.1694465350419,4.));
#3409=CARTESIAN_POINT('',(0.889666415794979,-79.5433889307008,3.));
#3410=CARTESIAN_POINT('',(-4.01080902459558,-50.1466711898151,3.));
#3411=CARTESIAN_POINT('Origin',(44.4833207897487,-57.1694465350419,3.));
#3412=CARTESIAN_POINT('',(0.889666415794979,-79.5433889307008,-3.));
#3413=CARTESIAN_POINT('',(0.889666415794979,-79.5433889307008,3.));
#3414=CARTESIAN_POINT('',(-4.01080902459558,-50.1466711898151,-3.));
#3415=CARTESIAN_POINT('Origin',(44.4833207897487,-57.1694465350419,-3.));
#3416=CARTESIAN_POINT('',(-4.01080902459558,-50.1466711898151,3.));
#3417=CARTESIAN_POINT('Origin',(44.4833207897487,-57.1694465350419,4.));
#3418=CARTESIAN_POINT('',(5.33799849476985,-77.260333584205,4.));
#3419=CARTESIAN_POINT('',(0.935261287824902,-50.8792546765288,4.));
#3420=CARTESIAN_POINT('Origin',(44.4833207897487,-57.1694465350419,4.));
#3421=CARTESIAN_POINT('',(5.33799849476985,-77.260333584205,3.));
#3422=CARTESIAN_POINT('',(5.33799849476985,-77.260333584205,4.));
#3423=CARTESIAN_POINT('',(0.935261287824902,-50.8792546765288,3.));
#3424=CARTESIAN_POINT('Origin',(44.4833207897487,-57.1694465350419,3.));
#3425=CARTESIAN_POINT('',(0.935261287824902,-50.8792546765288,4.));
#3426=CARTESIAN_POINT('Origin',(44.4833207897487,-57.1694465350419,4.));
#3427=CARTESIAN_POINT('',(6.93889390390723E-15,-80.,4.));
#3428=CARTESIAN_POINT('',(-5.,-50.0000000000001,4.));
#3429=CARTESIAN_POINT('Origin',(44.4833207897487,-57.1694465350419,4.));
#3430=CARTESIAN_POINT('',(-5.,-50.0000000000001,-4.));
#3431=CARTESIAN_POINT('',(-5.,-50.0000000000001,4.));
#3432=CARTESIAN_POINT('',(6.93889390390723E-15,-80.,-4.));
#3433=CARTESIAN_POINT('Origin',(44.4833207897487,-57.1694465350419,-4.));
#3434=CARTESIAN_POINT('',(6.93889390390723E-15,-80.,4.));
#3435=CARTESIAN_POINT('Origin',(44.4833207897487,-57.1694465350419,4.));
#3436=CARTESIAN_POINT('',(5.33799849476985,-77.260333584205,-3.));
#3437=CARTESIAN_POINT('',(0.935261287824902,-50.8792546765288,-3.));
#3438=CARTESIAN_POINT('Origin',(44.4833207897487,-57.1694465350419,-3.));
#3439=CARTESIAN_POINT('',(5.33799849476985,-77.260333584205,-4.));
#3440=CARTESIAN_POINT('',(5.33799849476985,-77.260333584205,4.));
#3441=CARTESIAN_POINT('',(0.935261287824902,-50.8792546765288,-4.));
#3442=CARTESIAN_POINT('Origin',(44.4833207897487,-57.1694465350419,-4.));
#3443=CARTESIAN_POINT('',(0.935261287824902,-50.8792546765288,4.));
#3444=CARTESIAN_POINT('Origin',(1.00000000000001,-14.5540683672724,4.));
#3445=CARTESIAN_POINT('',(1.00000000000001,-14.5540683672724,-3.));
#3446=CARTESIAN_POINT('',(6.00000000000001,-14.5540683672724,-3.));
#3447=CARTESIAN_POINT('',(1.00000000000001,-14.5540683672724,-3.));
#3448=CARTESIAN_POINT('',(1.00000000000001,-14.5540683672724,-4.));
#3449=CARTESIAN_POINT('',(1.00000000000001,-14.5540683672724,4.));
#3450=CARTESIAN_POINT('',(6.00000000000001,-14.5540683672724,-4.));
#3451=CARTESIAN_POINT('',(1.00000000000001,-14.5540683672724,-4.));
#3452=CARTESIAN_POINT('',(6.00000000000001,-14.5540683672724,4.));
#3453=CARTESIAN_POINT('Origin',(6.00000000000001,-14.5540683672724,4.));
#3454=CARTESIAN_POINT('',(4.98850765468119,0.338808764920716,-3.));
#3455=CARTESIAN_POINT('',(6.00000000000001,-14.5540683672724,-3.));
#3456=CARTESIAN_POINT('',(4.98850765468119,0.338808764920716,-4.));
#3457=CARTESIAN_POINT('',(6.00000000000001,-14.5540683672724,-4.));
#3458=CARTESIAN_POINT('',(4.98850765468119,0.338808764920716,4.));
#3459=CARTESIAN_POINT('Origin',(0.,0.,4.));
#3460=CARTESIAN_POINT('',(-4.99999999999999,6.12323399573676E-16,-3.));
#3461=CARTESIAN_POINT('Origin',(0.,0.,-3.));
#3462=CARTESIAN_POINT('',(-4.99999999999999,6.12323399573676E-16,-4.));
#3463=CARTESIAN_POINT('Origin',(0.,0.,-4.));
#3464=CARTESIAN_POINT('',(-4.99999999999999,6.12323399573676E-16,4.));
#3465=CARTESIAN_POINT('Origin',(-4.99999999999999,-20.,4.));
#3466=CARTESIAN_POINT('',(-4.99999999999999,-19.9623339466002,3.));
#3467=CARTESIAN_POINT('',(-4.99999999999999,-19.9623339466002,-3.));
#3468=CARTESIAN_POINT('',(-4.99999999999999,-19.9623339466002,-3.));
#3469=CARTESIAN_POINT('',(-4.99999999999999,-20.,-3.));
#3470=CARTESIAN_POINT('',(-4.99999999999999,-20.,-4.));
#3471=CARTESIAN_POINT('',(-4.99999999999999,-20.,-4.));
#3472=CARTESIAN_POINT('',(-4.99999999999999,-20.,4.));
#3473=CARTESIAN_POINT('',(-4.99999999999999,-20.,4.));
#3474=CARTESIAN_POINT('',(-4.99999999999999,6.12323399573676E-16,4.));
#3475=CARTESIAN_POINT('',(-4.99999999999999,-20.,4.));
#3476=CARTESIAN_POINT('',(-4.99999999999999,6.12323399573676E-16,3.));
#3477=CARTESIAN_POINT('',(-4.99999999999999,6.12323399573676E-16,4.));
#3478=CARTESIAN_POINT('',(-4.99999999999999,-20.,3.));
#3479=CARTESIAN_POINT('Origin',(0.,-80.,4.));
#3480=CARTESIAN_POINT('',(0.,-80.,-3.));
#3481=CARTESIAN_POINT('',(0.,-80.,3.));
#3482=CARTESIAN_POINT('',(0.,-80.,4.));
#3483=CARTESIAN_POINT('',(0.,-80.,-4.));
#3484=CARTESIAN_POINT('Origin',(-103.868599666426,-35.,4.));
#3485=CARTESIAN_POINT('',(1.,-19.5540683672724,-3.));
#3486=CARTESIAN_POINT('Origin',(-103.868599666426,-35.,-3.));
#3487=CARTESIAN_POINT('',(1.,-19.5540683672724,-4.));
#3488=CARTESIAN_POINT('Origin',(-103.868599666426,-35.,-4.));
#3489=CARTESIAN_POINT('',(1.,-19.5540683672724,4.));
#3490=CARTESIAN_POINT('Origin',(1.,-19.5540683672724,4.));
#3491=CARTESIAN_POINT('',(1.,-19.5540683672724,-3.));
#3492=CARTESIAN_POINT('',(1.,-19.5540683672724,-4.));
#3493=CARTESIAN_POINT('Origin',(1.00000000000001,-14.5540683672724,4.));
#3494=CARTESIAN_POINT('',(1.00000000000001,-14.5540683672724,4.));
#3495=CARTESIAN_POINT('',(1.00000000000001,-14.5540683672724,3.));
#3496=CARTESIAN_POINT('',(1.00000000000001,-14.5540683672724,4.));
#3497=CARTESIAN_POINT('',(6.00000000000001,-14.5540683672724,3.));
#3498=CARTESIAN_POINT('',(1.00000000000001,-14.5540683672724,3.));
#3499=CARTESIAN_POINT('',(6.00000000000001,-14.5540683672724,4.));
#3500=CARTESIAN_POINT('',(6.00000000000001,-14.5540683672724,4.));
#3501=CARTESIAN_POINT('',(1.00000000000001,-14.5540683672724,4.));
#3502=CARTESIAN_POINT('Origin',(6.00000000000001,-14.5540683672724,4.));
#3503=CARTESIAN_POINT('',(4.98850765468119,0.338808764920716,3.));
#3504=CARTESIAN_POINT('',(6.00000000000001,-14.5540683672724,3.));
#3505=CARTESIAN_POINT('',(4.98850765468119,0.338808764920716,4.));
#3506=CARTESIAN_POINT('',(4.98850765468119,0.338808764920716,4.));
#3507=CARTESIAN_POINT('',(6.00000000000001,-14.5540683672724,4.));
#3508=CARTESIAN_POINT('Origin',(0.,0.,4.));
#3509=CARTESIAN_POINT('Origin',(0.,0.,3.));
#3510=CARTESIAN_POINT('Origin',(0.,0.,4.));
#3511=CARTESIAN_POINT('Origin',(-103.868599666426,-35.,4.));
#3512=CARTESIAN_POINT('Origin',(-103.868599666426,-35.,-4.));
#3513=CARTESIAN_POINT('Origin',(-103.868599666426,-35.,4.));
#3514=CARTESIAN_POINT('Origin',(-103.868599666426,-35.,4.));
#3515=CARTESIAN_POINT('',(1.,-19.5540683672724,3.));
#3516=CARTESIAN_POINT('Origin',(-103.868599666426,-35.,3.));
#3517=CARTESIAN_POINT('',(1.,-19.5540683672724,4.));
#3518=CARTESIAN_POINT('',(1.,-19.5540683672724,4.));
#3519=CARTESIAN_POINT('Origin',(-103.868599666426,-35.,4.));
#3520=CARTESIAN_POINT('Origin',(1.,-19.5540683672724,4.));
#3521=CARTESIAN_POINT('',(1.,-19.5540683672724,3.));
#3522=CARTESIAN_POINT('',(1.,-19.5540683672724,4.));
#3523=CARTESIAN_POINT('Origin',(0.,0.,4.));
#3524=CARTESIAN_POINT('Origin',(0.,0.,-4.));
#3525=CARTESIAN_POINT('Origin',(-103.868599666426,-35.,4.));
#3526=CARTESIAN_POINT('',(-4.00562885738096,-19.8875196876281,-3.));
#3527=CARTESIAN_POINT('Origin',(-103.868599666426,-35.,-3.));
#3528=CARTESIAN_POINT('',(-4.00562885738096,-19.8875196876281,3.));
#3529=CARTESIAN_POINT('',(-4.00562885738094,-19.8875196876281,4.));
#3530=CARTESIAN_POINT('Origin',(-103.868599666426,-35.,3.));
#3531=CARTESIAN_POINT('Origin',(0.,0.,3.));
#3532=CARTESIAN_POINT('Origin',(-4.49999999999999,-19.9623339466002,3.));
#3533=CARTESIAN_POINT('Origin',(0.,0.,-3.));
#3534=CARTESIAN_POINT('Origin',(-4.49999999999999,-19.9623339466002,-3.));
#3535=CARTESIAN_POINT('Origin',(-4.49999999999999,-19.9623339466002,4.));
#3536=CARTESIAN_POINT('Origin',(0.,-10.,-3.5));
#3537=CARTESIAN_POINT('Origin',(0.,-10.,3.5));
#9547=UNCERTAINTY_MEASURE_WITH_UNIT(LENGTH_MEASURE(0.01),#9562,
'DISTANCE_ACCURACY_VALUE',
'Maximum model space distance between geometric entities at asserted c
onnectivities');
#9553=UNCERTAINTY_MEASURE_WITH_UNIT(LENGTH_MEASURE(0.01),#9562,
'DISTANCE_ACCURACY_VALUE',
'Maximum model space distance between geometric entities at asserted c
onnectivities');
#9555=(
GEOMETRIC_REPRESENTATION_CONTEXT(3)
GLOBAL_UNCERTAINTY_ASSIGNED_CONTEXT((#9547))
GLOBAL_UNIT_ASSIGNED_CONTEXT((#9562,#9564,#9565))
REPRESENTATION_CONTEXT('','3D')
);
#9561=(
GEOMETRIC_REPRESENTATION_CONTEXT(3)
GLOBAL_UNCERTAINTY_ASSIGNED_CONTEXT((#9553))
GLOBAL_UNIT_ASSIGNED_CONTEXT((#9562,#9564,#9565))
REPRESENTATION_CONTEXT('','3D')
);
#9562=(
LENGTH_UNIT()
NAMED_UNIT(*)
SI_UNIT(.MILLI.,.METRE.)
);
#9564=(
NAMED_UNIT(*)
PLANE_ANGLE_UNIT()
SI_UNIT($,.RADIAN.)
);
#9565=(
NAMED_UNIT(*)
SI_UNIT($,.STERADIAN.)
SOLID_ANGLE_UNIT()
);
#9567=SHAPE_DEFINITION_REPRESENTATION(#9574,#9587);
#9574=PRODUCT_DEFINITION_SHAPE('',$,#9595);
#9587=SHAPE_REPRESENTATION('',(#2479),#9555);
#9593=PRODUCT_DEFINITION_CONTEXT('part definition',#9616,'design');
#9595=PRODUCT_DEFINITION('Handle','Handle',#9602,#9593);
#9602=PRODUCT_DEFINITION_FORMATION('',$,#9619);
#9616=APPLICATION_CONTEXT(
'Core Data for Automotive Mechanical Design Process');
#9617=PRODUCT_CONTEXT('part definition',#9616,'mechanical');
#9619=PRODUCT('Handle','Handle',$,(#9617));
#9626=PRESENTATION_STYLE_ASSIGNMENT((#9631));
#9631=SURFACE_STYLE_USAGE(.BOTH.,#9636);
#9636=SURFACE_SIDE_STYLE('',(#9641));
#9641=SURFACE_STYLE_FILL_AREA(#9646);
#9646=FILL_AREA_STYLE('Opaque(61,176,222)',(#9651));
#9651=FILL_AREA_STYLE_COLOUR('Opaque(61,176,222)',#9656);
#9656=COLOUR_RGB('Opaque(61,176,222)',0.23921568627451,0.690196078431373,
0.870588235294118);
ENDSEC;
END-ISO-10303-21;
